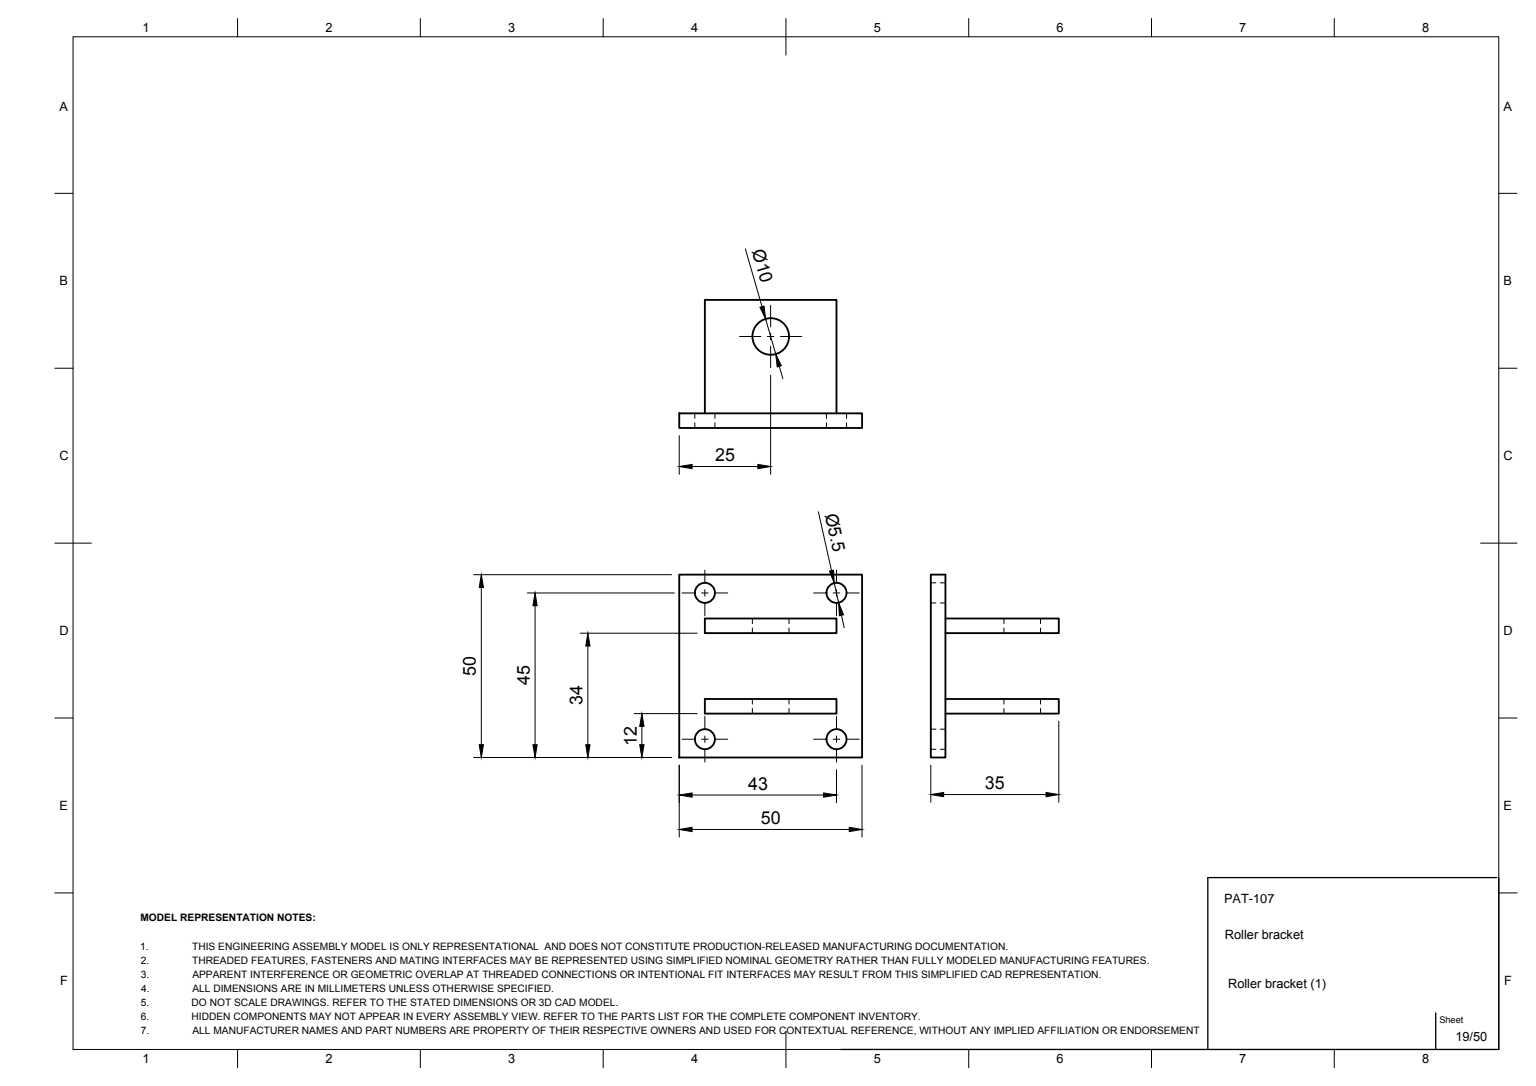
ISO-10303-21;
HEADER;
/* Generated by software containing ST-Developer
 * from STEP Tools, Inc. (www.steptools.com) 
 */

FILE_DESCRIPTION(
/* description */ ('Turntable on roller ring'),
/* implementation_level */ '2;1');

FILE_NAME(
/* name */ 'Roller bracket (1).step',
/* time_stamp */ '2026-10-28T03:23:59-07:00',
/* author */ (''),
/* organization */ (''),
/* preprocessor_version */ 'ST-DEVELOPER v20.2',
/* originating_system */ 'Autodesk Translation Framework v15.17.0.0',
/* authorisation */ '');

FILE_SCHEMA (('AUTOMOTIVE_DESIGN { 1 0 10303 214 3 1 1 }'));
ENDSEC;

DATA;
#10=MECHANICAL_DESIGN_GEOMETRIC_PRESENTATION_REPRESENTATION('',(#647),#16281);
#528=SHAPE_REPRESENTATION_RELATIONSHIP('SRR','None',#16546,#583);
#583=ADVANCED_BREP_SHAPE_REPRESENTATION('',(#717),#16240);
#647=STYLED_ITEM('',(#16911),#717);
#717=MANIFOLD_SOLID_BREP('Body1',#8390);
#889=FACE_BOUND('',#2148,.T.);
#890=FACE_BOUND('',#2150,.T.);
#891=FACE_BOUND('',#2155,.T.);
#892=FACE_BOUND('',#2157,.T.);
#893=FACE_BOUND('',#2163,.T.);
#894=FACE_BOUND('',#2164,.T.);
#895=FACE_BOUND('',#2165,.T.);
#896=FACE_BOUND('',#2166,.T.);
#897=FACE_BOUND('',#2167,.T.);
#898=FACE_BOUND('',#2168,.T.);
#899=FACE_BOUND('',#2170,.T.);
#900=FACE_BOUND('',#2171,.T.);
#901=FACE_BOUND('',#2172,.T.);
#902=FACE_BOUND('',#2173,.T.);
#1109=PLANE('',#9629);
#1110=PLANE('',#9630);
#1111=PLANE('',#9631);
#1112=PLANE('',#9632);
#1113=PLANE('',#9633);
#1114=PLANE('',#9634);
#1115=PLANE('',#9635);
#1116=PLANE('',#9636);
#1117=PLANE('',#9637);
#1118=PLANE('',#9638);
#1119=PLANE('',#9639);
#1120=PLANE('',#9640);
#1121=PLANE('',#9641);
#1122=PLANE('',#9642);
#1123=PLANE('',#9643);
#1124=PLANE('',#9644);
#1501=FACE_OUTER_BOUND('',#2138,.T.);
#1502=FACE_OUTER_BOUND('',#2139,.T.);
#1503=FACE_OUTER_BOUND('',#2140,.T.);
#1504=FACE_OUTER_BOUND('',#2141,.T.);
#1505=FACE_OUTER_BOUND('',#2142,.T.);
#1506=FACE_OUTER_BOUND('',#2143,.T.);
#1507=FACE_OUTER_BOUND('',#2144,.T.);
#1508=FACE_OUTER_BOUND('',#2145,.T.);
#1509=FACE_OUTER_BOUND('',#2146,.T.);
#1510=FACE_OUTER_BOUND('',#2147,.T.);
#1511=FACE_OUTER_BOUND('',#2149,.T.);
#1512=FACE_OUTER_BOUND('',#2151,.T.);
#1513=FACE_OUTER_BOUND('',#2152,.T.);
#1514=FACE_OUTER_BOUND('',#2153,.T.);
#1515=FACE_OUTER_BOUND('',#2154,.T.);
#1516=FACE_OUTER_BOUND('',#2156,.T.);
#1517=FACE_OUTER_BOUND('',#2158,.T.);
#1518=FACE_OUTER_BOUND('',#2159,.T.);
#1519=FACE_OUTER_BOUND('',#2160,.T.);
#1520=FACE_OUTER_BOUND('',#2161,.T.);
#1521=FACE_OUTER_BOUND('',#2162,.T.);
#1522=FACE_OUTER_BOUND('',#2169,.T.);
#2138=EDGE_LOOP('',(#6707,#6708,#6709,#6710));
#2139=EDGE_LOOP('',(#6711,#6712,#6713,#6714));
#2140=EDGE_LOOP('',(#6715,#6716,#6717,#6718));
#2141=EDGE_LOOP('',(#6719,#6720,#6721,#6722));
#2142=EDGE_LOOP('',(#6723,#6724,#6725,#6726));
#2143=EDGE_LOOP('',(#6727,#6728,#6729,#6730));
#2144=EDGE_LOOP('',(#6731,#6732,#6733,#6734));
#2145=EDGE_LOOP('',(#6735,#6736,#6737,#6738));
#2146=EDGE_LOOP('',(#6739,#6740,#6741,#6742));
#2147=EDGE_LOOP('',(#6743,#6744,#6745,#6746));
#2148=EDGE_LOOP('',(#6747));
#2149=EDGE_LOOP('',(#6748,#6749,#6750,#6751));
#2150=EDGE_LOOP('',(#6752));
#2151=EDGE_LOOP('',(#6753,#6754,#6755,#6756));
#2152=EDGE_LOOP('',(#6757,#6758,#6759,#6760));
#2153=EDGE_LOOP('',(#6761,#6762,#6763,#6764));
#2154=EDGE_LOOP('',(#6765,#6766,#6767,#6768));
#2155=EDGE_LOOP('',(#6769));
#2156=EDGE_LOOP('',(#6770,#6771,#6772,#6773));
#2157=EDGE_LOOP('',(#6774));
#2158=EDGE_LOOP('',(#6775,#6776,#6777,#6778));
#2159=EDGE_LOOP('',(#6779,#6780,#6781,#6782));
#2160=EDGE_LOOP('',(#6783,#6784,#6785,#6786));
#2161=EDGE_LOOP('',(#6787,#6788,#6789,#6790));
#2162=EDGE_LOOP('',(#6791,#6792,#6793,#6794));
#2163=EDGE_LOOP('',(#6795,#6796,#6797,#6798));
#2164=EDGE_LOOP('',(#6799,#6800,#6801,#6802));
#2165=EDGE_LOOP('',(#6803));
#2166=EDGE_LOOP('',(#6804));
#2167=EDGE_LOOP('',(#6805));
#2168=EDGE_LOOP('',(#6806));
#2169=EDGE_LOOP('',(#6807,#6808,#6809,#6810));
#2170=EDGE_LOOP('',(#6811));
#2171=EDGE_LOOP('',(#6812));
#2172=EDGE_LOOP('',(#6813));
#2173=EDGE_LOOP('',(#6814));
#2737=LINE('',#14636,#3220);
#2738=LINE('',#14642,#3221);
#2739=LINE('',#14648,#3222);
#2740=LINE('',#14654,#3223);
#2741=LINE('',#14660,#3224);
#2742=LINE('',#14666,#3225);
#2743=LINE('',#14671,#3226);
#2744=LINE('',#14673,#3227);
#2745=LINE('',#14675,#3228);
#2746=LINE('',#14676,#3229);
#2747=LINE('',#14680,#3230);
#2748=LINE('',#14682,#3231);
#2749=LINE('',#14684,#3232);
#2750=LINE('',#14685,#3233);
#2751=LINE('',#14687,#3234);
#2752=LINE('',#14688,#3235);
#2753=LINE('',#14690,#3236);
#2754=LINE('',#14692,#3237);
#2755=LINE('',#14696,#3238);
#2756=LINE('',#14698,#3239);
#2757=LINE('',#14700,#3240);
#2758=LINE('',#14701,#3241);
#2759=LINE('',#14705,#3242);
#2760=LINE('',#14707,#3243);
#2761=LINE('',#14709,#3244);
#2762=LINE('',#14710,#3245);
#2763=LINE('',#14712,#3246);
#2764=LINE('',#14713,#3247);
#2765=LINE('',#14715,#3248);
#2766=LINE('',#14717,#3249);
#2767=LINE('',#14721,#3250);
#2768=LINE('',#14723,#3251);
#2769=LINE('',#14725,#3252);
#2770=LINE('',#14726,#3253);
#2771=LINE('',#14729,#3254);
#2772=LINE('',#14731,#3255);
#2773=LINE('',#14732,#3256);
#2774=LINE('',#14735,#3257);
#2775=LINE('',#14737,#3258);
#2776=LINE('',#14738,#3259);
#2777=LINE('',#14740,#3260);
#2778=LINE('',#14741,#3261);
#3220=VECTOR('',#11590,0.275);
#3221=VECTOR('',#11597,0.275);
#3222=VECTOR('',#11604,0.275);
#3223=VECTOR('',#11611,0.275);
#3224=VECTOR('',#11618,0.5);
#3225=VECTOR('',#11625,0.5);
#3226=VECTOR('',#11630,1.);
#3227=VECTOR('',#11631,1.);
#3228=VECTOR('',#11632,1.);
#3229=VECTOR('',#11633,1.);
#3230=VECTOR('',#11636,1.);
#3231=VECTOR('',#11637,1.);
#3232=VECTOR('',#11638,1.);
#3233=VECTOR('',#11639,1.);
#3234=VECTOR('',#11642,1.);
#3235=VECTOR('',#11643,1.);
#3236=VECTOR('',#11646,1.);
#3237=VECTOR('',#11649,1.);
#3238=VECTOR('',#11652,1.);
#3239=VECTOR('',#11653,1.);
#3240=VECTOR('',#11654,1.);
#3241=VECTOR('',#11655,1.);
#3242=VECTOR('',#11658,1.);
#3243=VECTOR('',#11659,1.);
#3244=VECTOR('',#11660,1.);
#3245=VECTOR('',#11661,1.);
#3246=VECTOR('',#11664,1.);
#3247=VECTOR('',#11665,1.);
#3248=VECTOR('',#11668,1.);
#3249=VECTOR('',#11671,1.);
#3250=VECTOR('',#11674,1.);
#3251=VECTOR('',#11675,1.);
#3252=VECTOR('',#11676,1.);
#3253=VECTOR('',#11677,1.);
#3254=VECTOR('',#11680,1.);
#3255=VECTOR('',#11681,1.);
#3256=VECTOR('',#11682,1.);
#3257=VECTOR('',#11685,1.);
#3258=VECTOR('',#11686,1.);
#3259=VECTOR('',#11687,1.);
#3260=VECTOR('',#11690,1.);
#3261=VECTOR('',#11691,1.);
#3725=CIRCLE('',#9612,0.275);
#3726=CIRCLE('',#9613,0.275);
#3727=CIRCLE('',#9615,0.275);
#3728=CIRCLE('',#9616,0.275);
#3729=CIRCLE('',#9618,0.275);
#3730=CIRCLE('',#9619,0.275);
#3731=CIRCLE('',#9621,0.275);
#3732=CIRCLE('',#9622,0.275);
#3733=CIRCLE('',#9624,0.5);
#3734=CIRCLE('',#9625,0.5);
#3735=CIRCLE('',#9627,0.5);
#3736=CIRCLE('',#9628,0.5);
#4305=VERTEX_POINT('',#14633);
#4306=VERTEX_POINT('',#14635);
#4307=VERTEX_POINT('',#14639);
#4308=VERTEX_POINT('',#14641);
#4309=VERTEX_POINT('',#14645);
#4310=VERTEX_POINT('',#14647);
#4311=VERTEX_POINT('',#14651);
#4312=VERTEX_POINT('',#14653);
#4313=VERTEX_POINT('',#14657);
#4314=VERTEX_POINT('',#14659);
#4315=VERTEX_POINT('',#14663);
#4316=VERTEX_POINT('',#14665);
#4317=VERTEX_POINT('',#14669);
#4318=VERTEX_POINT('',#14670);
#4319=VERTEX_POINT('',#14672);
#4320=VERTEX_POINT('',#14674);
#4321=VERTEX_POINT('',#14678);
#4322=VERTEX_POINT('',#14679);
#4323=VERTEX_POINT('',#14681);
#4324=VERTEX_POINT('',#14683);
#4325=VERTEX_POINT('',#14694);
#4326=VERTEX_POINT('',#14695);
#4327=VERTEX_POINT('',#14697);
#4328=VERTEX_POINT('',#14699);
#4329=VERTEX_POINT('',#14703);
#4330=VERTEX_POINT('',#14704);
#4331=VERTEX_POINT('',#14706);
#4332=VERTEX_POINT('',#14708);
#4333=VERTEX_POINT('',#14719);
#4334=VERTEX_POINT('',#14720);
#4335=VERTEX_POINT('',#14722);
#4336=VERTEX_POINT('',#14724);
#4337=VERTEX_POINT('',#14728);
#4338=VERTEX_POINT('',#14730);
#4339=VERTEX_POINT('',#14734);
#4340=VERTEX_POINT('',#14736);
#5164=EDGE_CURVE('',#4305,#4305,#3725,.T.);
#5165=EDGE_CURVE('',#4305,#4306,#2737,.T.);
#5166=EDGE_CURVE('',#4306,#4306,#3726,.T.);
#5167=EDGE_CURVE('',#4307,#4307,#3727,.T.);
#5168=EDGE_CURVE('',#4307,#4308,#2738,.T.);
#5169=EDGE_CURVE('',#4308,#4308,#3728,.T.);
#5170=EDGE_CURVE('',#4309,#4309,#3729,.T.);
#5171=EDGE_CURVE('',#4309,#4310,#2739,.T.);
#5172=EDGE_CURVE('',#4310,#4310,#3730,.T.);
#5173=EDGE_CURVE('',#4311,#4311,#3731,.T.);
#5174=EDGE_CURVE('',#4311,#4312,#2740,.T.);
#5175=EDGE_CURVE('',#4312,#4312,#3732,.T.);
#5176=EDGE_CURVE('',#4313,#4313,#3733,.T.);
#5177=EDGE_CURVE('',#4313,#4314,#2741,.T.);
#5178=EDGE_CURVE('',#4314,#4314,#3734,.T.);
#5179=EDGE_CURVE('',#4315,#4315,#3735,.T.);
#5180=EDGE_CURVE('',#4315,#4316,#2742,.T.);
#5181=EDGE_CURVE('',#4316,#4316,#3736,.T.);
#5182=EDGE_CURVE('',#4317,#4318,#2743,.T.);
#5183=EDGE_CURVE('',#4317,#4319,#2744,.T.);
#5184=EDGE_CURVE('',#4320,#4319,#2745,.T.);
#5185=EDGE_CURVE('',#4318,#4320,#2746,.T.);
#5186=EDGE_CURVE('',#4321,#4322,#2747,.T.);
#5187=EDGE_CURVE('',#4323,#4321,#2748,.T.);
#5188=EDGE_CURVE('',#4324,#4323,#2749,.T.);
#5189=EDGE_CURVE('',#4322,#4324,#2750,.T.);
#5190=EDGE_CURVE('',#4322,#4317,#2751,.T.);
#5191=EDGE_CURVE('',#4319,#4324,#2752,.T.);
#5192=EDGE_CURVE('',#4320,#4323,#2753,.T.);
#5193=EDGE_CURVE('',#4321,#4318,#2754,.T.);
#5194=EDGE_CURVE('',#4325,#4326,#2755,.T.);
#5195=EDGE_CURVE('',#4325,#4327,#2756,.T.);
#5196=EDGE_CURVE('',#4328,#4327,#2757,.T.);
#5197=EDGE_CURVE('',#4326,#4328,#2758,.T.);
#5198=EDGE_CURVE('',#4329,#4330,#2759,.T.);
#5199=EDGE_CURVE('',#4331,#4329,#2760,.T.);
#5200=EDGE_CURVE('',#4332,#4331,#2761,.T.);
#5201=EDGE_CURVE('',#4330,#4332,#2762,.T.);
#5202=EDGE_CURVE('',#4330,#4325,#2763,.T.);
#5203=EDGE_CURVE('',#4327,#4332,#2764,.T.);
#5204=EDGE_CURVE('',#4328,#4331,#2765,.T.);
#5205=EDGE_CURVE('',#4329,#4326,#2766,.T.);
#5206=EDGE_CURVE('',#4333,#4334,#2767,.T.);
#5207=EDGE_CURVE('',#4334,#4335,#2768,.T.);
#5208=EDGE_CURVE('',#4336,#4335,#2769,.T.);
#5209=EDGE_CURVE('',#4333,#4336,#2770,.T.);
#5210=EDGE_CURVE('',#4337,#4333,#2771,.T.);
#5211=EDGE_CURVE('',#4338,#4336,#2772,.T.);
#5212=EDGE_CURVE('',#4337,#4338,#2773,.T.);
#5213=EDGE_CURVE('',#4339,#4337,#2774,.T.);
#5214=EDGE_CURVE('',#4340,#4338,#2775,.T.);
#5215=EDGE_CURVE('',#4339,#4340,#2776,.T.);
#5216=EDGE_CURVE('',#4334,#4339,#2777,.T.);
#5217=EDGE_CURVE('',#4335,#4340,#2778,.T.);
#6707=ORIENTED_EDGE('',*,*,#5164,.F.);
#6708=ORIENTED_EDGE('',*,*,#5165,.T.);
#6709=ORIENTED_EDGE('',*,*,#5166,.F.);
#6710=ORIENTED_EDGE('',*,*,#5165,.F.);
#6711=ORIENTED_EDGE('',*,*,#5167,.F.);
#6712=ORIENTED_EDGE('',*,*,#5168,.T.);
#6713=ORIENTED_EDGE('',*,*,#5169,.F.);
#6714=ORIENTED_EDGE('',*,*,#5168,.F.);
#6715=ORIENTED_EDGE('',*,*,#5170,.F.);
#6716=ORIENTED_EDGE('',*,*,#5171,.T.);
#6717=ORIENTED_EDGE('',*,*,#5172,.F.);
#6718=ORIENTED_EDGE('',*,*,#5171,.F.);
#6719=ORIENTED_EDGE('',*,*,#5173,.F.);
#6720=ORIENTED_EDGE('',*,*,#5174,.T.);
#6721=ORIENTED_EDGE('',*,*,#5175,.F.);
#6722=ORIENTED_EDGE('',*,*,#5174,.F.);
#6723=ORIENTED_EDGE('',*,*,#5176,.F.);
#6724=ORIENTED_EDGE('',*,*,#5177,.T.);
#6725=ORIENTED_EDGE('',*,*,#5178,.F.);
#6726=ORIENTED_EDGE('',*,*,#5177,.F.);
#6727=ORIENTED_EDGE('',*,*,#5179,.F.);
#6728=ORIENTED_EDGE('',*,*,#5180,.T.);
#6729=ORIENTED_EDGE('',*,*,#5181,.F.);
#6730=ORIENTED_EDGE('',*,*,#5180,.F.);
#6731=ORIENTED_EDGE('',*,*,#5182,.F.);
#6732=ORIENTED_EDGE('',*,*,#5183,.T.);
#6733=ORIENTED_EDGE('',*,*,#5184,.F.);
#6734=ORIENTED_EDGE('',*,*,#5185,.F.);
#6735=ORIENTED_EDGE('',*,*,#5186,.F.);
#6736=ORIENTED_EDGE('',*,*,#5187,.F.);
#6737=ORIENTED_EDGE('',*,*,#5188,.F.);
#6738=ORIENTED_EDGE('',*,*,#5189,.F.);
#6739=ORIENTED_EDGE('',*,*,#5190,.F.);
#6740=ORIENTED_EDGE('',*,*,#5189,.T.);
#6741=ORIENTED_EDGE('',*,*,#5191,.F.);
#6742=ORIENTED_EDGE('',*,*,#5183,.F.);
#6743=ORIENTED_EDGE('',*,*,#5191,.T.);
#6744=ORIENTED_EDGE('',*,*,#5188,.T.);
#6745=ORIENTED_EDGE('',*,*,#5192,.F.);
#6746=ORIENTED_EDGE('',*,*,#5184,.T.);
#6747=ORIENTED_EDGE('',*,*,#5181,.T.);
#6748=ORIENTED_EDGE('',*,*,#5190,.T.);
#6749=ORIENTED_EDGE('',*,*,#5182,.T.);
#6750=ORIENTED_EDGE('',*,*,#5193,.F.);
#6751=ORIENTED_EDGE('',*,*,#5186,.T.);
#6752=ORIENTED_EDGE('',*,*,#5179,.T.);
#6753=ORIENTED_EDGE('',*,*,#5194,.F.);
#6754=ORIENTED_EDGE('',*,*,#5195,.T.);
#6755=ORIENTED_EDGE('',*,*,#5196,.F.);
#6756=ORIENTED_EDGE('',*,*,#5197,.F.);
#6757=ORIENTED_EDGE('',*,*,#5198,.F.);
#6758=ORIENTED_EDGE('',*,*,#5199,.F.);
#6759=ORIENTED_EDGE('',*,*,#5200,.F.);
#6760=ORIENTED_EDGE('',*,*,#5201,.F.);
#6761=ORIENTED_EDGE('',*,*,#5202,.F.);
#6762=ORIENTED_EDGE('',*,*,#5201,.T.);
#6763=ORIENTED_EDGE('',*,*,#5203,.F.);
#6764=ORIENTED_EDGE('',*,*,#5195,.F.);
#6765=ORIENTED_EDGE('',*,*,#5203,.T.);
#6766=ORIENTED_EDGE('',*,*,#5200,.T.);
#6767=ORIENTED_EDGE('',*,*,#5204,.F.);
#6768=ORIENTED_EDGE('',*,*,#5196,.T.);
#6769=ORIENTED_EDGE('',*,*,#5178,.T.);
#6770=ORIENTED_EDGE('',*,*,#5202,.T.);
#6771=ORIENTED_EDGE('',*,*,#5194,.T.);
#6772=ORIENTED_EDGE('',*,*,#5205,.F.);
#6773=ORIENTED_EDGE('',*,*,#5198,.T.);
#6774=ORIENTED_EDGE('',*,*,#5176,.T.);
#6775=ORIENTED_EDGE('',*,*,#5206,.T.);
#6776=ORIENTED_EDGE('',*,*,#5207,.T.);
#6777=ORIENTED_EDGE('',*,*,#5208,.F.);
#6778=ORIENTED_EDGE('',*,*,#5209,.F.);
#6779=ORIENTED_EDGE('',*,*,#5210,.T.);
#6780=ORIENTED_EDGE('',*,*,#5209,.T.);
#6781=ORIENTED_EDGE('',*,*,#5211,.F.);
#6782=ORIENTED_EDGE('',*,*,#5212,.F.);
#6783=ORIENTED_EDGE('',*,*,#5213,.T.);
#6784=ORIENTED_EDGE('',*,*,#5212,.T.);
#6785=ORIENTED_EDGE('',*,*,#5214,.F.);
#6786=ORIENTED_EDGE('',*,*,#5215,.F.);
#6787=ORIENTED_EDGE('',*,*,#5216,.T.);
#6788=ORIENTED_EDGE('',*,*,#5215,.T.);
#6789=ORIENTED_EDGE('',*,*,#5217,.F.);
#6790=ORIENTED_EDGE('',*,*,#5207,.F.);
#6791=ORIENTED_EDGE('',*,*,#5217,.T.);
#6792=ORIENTED_EDGE('',*,*,#5214,.T.);
#6793=ORIENTED_EDGE('',*,*,#5211,.T.);
#6794=ORIENTED_EDGE('',*,*,#5208,.T.);
#6795=ORIENTED_EDGE('',*,*,#5199,.T.);
#6796=ORIENTED_EDGE('',*,*,#5205,.T.);
#6797=ORIENTED_EDGE('',*,*,#5197,.T.);
#6798=ORIENTED_EDGE('',*,*,#5204,.T.);
#6799=ORIENTED_EDGE('',*,*,#5187,.T.);
#6800=ORIENTED_EDGE('',*,*,#5193,.T.);
#6801=ORIENTED_EDGE('',*,*,#5185,.T.);
#6802=ORIENTED_EDGE('',*,*,#5192,.T.);
#6803=ORIENTED_EDGE('',*,*,#5175,.T.);
#6804=ORIENTED_EDGE('',*,*,#5172,.T.);
#6805=ORIENTED_EDGE('',*,*,#5169,.T.);
#6806=ORIENTED_EDGE('',*,*,#5166,.T.);
#6807=ORIENTED_EDGE('',*,*,#5216,.F.);
#6808=ORIENTED_EDGE('',*,*,#5206,.F.);
#6809=ORIENTED_EDGE('',*,*,#5210,.F.);
#6810=ORIENTED_EDGE('',*,*,#5213,.F.);
#6811=ORIENTED_EDGE('',*,*,#5164,.T.);
#6812=ORIENTED_EDGE('',*,*,#5167,.T.);
#6813=ORIENTED_EDGE('',*,*,#5170,.T.);
#6814=ORIENTED_EDGE('',*,*,#5173,.T.);
#7768=CYLINDRICAL_SURFACE('',#9611,0.275);
#7769=CYLINDRICAL_SURFACE('',#9614,0.275);
#7770=CYLINDRICAL_SURFACE('',#9617,0.275);
#7771=CYLINDRICAL_SURFACE('',#9620,0.275);
#7772=CYLINDRICAL_SURFACE('',#9623,0.5);
#7773=CYLINDRICAL_SURFACE('',#9626,0.5);
#8104=ADVANCED_FACE('',(#1501),#7768,.F.);
#8105=ADVANCED_FACE('',(#1502),#7769,.F.);
#8106=ADVANCED_FACE('',(#1503),#7770,.F.);
#8107=ADVANCED_FACE('',(#1504),#7771,.F.);
#8108=ADVANCED_FACE('',(#1505),#7772,.F.);
#8109=ADVANCED_FACE('',(#1506),#7773,.F.);
#8110=ADVANCED_FACE('',(#1507),#1109,.T.);
#8111=ADVANCED_FACE('',(#1508),#1110,.T.);
#8112=ADVANCED_FACE('',(#1509),#1111,.T.);
#8113=ADVANCED_FACE('',(#1510,#889),#1112,.T.);
#8114=ADVANCED_FACE('',(#1511,#890),#1113,.F.);
#8115=ADVANCED_FACE('',(#1512),#1114,.T.);
#8116=ADVANCED_FACE('',(#1513),#1115,.T.);
#8117=ADVANCED_FACE('',(#1514),#1116,.T.);
#8118=ADVANCED_FACE('',(#1515,#891),#1117,.T.);
#8119=ADVANCED_FACE('',(#1516,#892),#1118,.F.);
#8120=ADVANCED_FACE('',(#1517),#1119,.T.);
#8121=ADVANCED_FACE('',(#1518),#1120,.T.);
#8122=ADVANCED_FACE('',(#1519),#1121,.T.);
#8123=ADVANCED_FACE('',(#1520),#1122,.T.);
#8124=ADVANCED_FACE('',(#1521,#893,#894,#895,#896,#897,#898),#1123,.T.);
#8125=ADVANCED_FACE('',(#1522,#899,#900,#901,#902),#1124,.F.);
#8390=CLOSED_SHELL('',(#8104,#8105,#8106,#8107,#8108,#8109,#8110,#8111,
#8112,#8113,#8114,#8115,#8116,#8117,#8118,#8119,#8120,#8121,#8122,#8123,
#8124,#8125));
#9610=AXIS2_PLACEMENT_3D('',#14631,#11584,#11585);
#9611=AXIS2_PLACEMENT_3D('',#14632,#11586,#11587);
#9612=AXIS2_PLACEMENT_3D('',#14634,#11588,#11589);
#9613=AXIS2_PLACEMENT_3D('',#14637,#11591,#11592);
#9614=AXIS2_PLACEMENT_3D('',#14638,#11593,#11594);
#9615=AXIS2_PLACEMENT_3D('',#14640,#11595,#11596);
#9616=AXIS2_PLACEMENT_3D('',#14643,#11598,#11599);
#9617=AXIS2_PLACEMENT_3D('',#14644,#11600,#11601);
#9618=AXIS2_PLACEMENT_3D('',#14646,#11602,#11603);
#9619=AXIS2_PLACEMENT_3D('',#14649,#11605,#11606);
#9620=AXIS2_PLACEMENT_3D('',#14650,#11607,#11608);
#9621=AXIS2_PLACEMENT_3D('',#14652,#11609,#11610);
#9622=AXIS2_PLACEMENT_3D('',#14655,#11612,#11613);
#9623=AXIS2_PLACEMENT_3D('',#14656,#11614,#11615);
#9624=AXIS2_PLACEMENT_3D('',#14658,#11616,#11617);
#9625=AXIS2_PLACEMENT_3D('',#14661,#11619,#11620);
#9626=AXIS2_PLACEMENT_3D('',#14662,#11621,#11622);
#9627=AXIS2_PLACEMENT_3D('',#14664,#11623,#11624);
#9628=AXIS2_PLACEMENT_3D('',#14667,#11626,#11627);
#9629=AXIS2_PLACEMENT_3D('',#14668,#11628,#11629);
#9630=AXIS2_PLACEMENT_3D('',#14677,#11634,#11635);
#9631=AXIS2_PLACEMENT_3D('',#14686,#11640,#11641);
#9632=AXIS2_PLACEMENT_3D('',#14689,#11644,#11645);
#9633=AXIS2_PLACEMENT_3D('',#14691,#11647,#11648);
#9634=AXIS2_PLACEMENT_3D('',#14693,#11650,#11651);
#9635=AXIS2_PLACEMENT_3D('',#14702,#11656,#11657);
#9636=AXIS2_PLACEMENT_3D('',#14711,#11662,#11663);
#9637=AXIS2_PLACEMENT_3D('',#14714,#11666,#11667);
#9638=AXIS2_PLACEMENT_3D('',#14716,#11669,#11670);
#9639=AXIS2_PLACEMENT_3D('',#14718,#11672,#11673);
#9640=AXIS2_PLACEMENT_3D('',#14727,#11678,#11679);
#9641=AXIS2_PLACEMENT_3D('',#14733,#11683,#11684);
#9642=AXIS2_PLACEMENT_3D('',#14739,#11688,#11689);
#9643=AXIS2_PLACEMENT_3D('',#14742,#11692,#11693);
#9644=AXIS2_PLACEMENT_3D('',#14743,#11694,#11695);
#11584=DIRECTION('axis',(0.,0.,1.));
#11585=DIRECTION('refdir',(1.,0.,0.));
#11586=DIRECTION('center_axis',(0.,0.,1.));
#11587=DIRECTION('ref_axis',(1.,0.,0.));
#11588=DIRECTION('center_axis',(0.,0.,1.));
#11589=DIRECTION('ref_axis',(1.,0.,0.));
#11590=DIRECTION('',(0.,0.,1.));
#11591=DIRECTION('center_axis',(0.,0.,-1.));
#11592=DIRECTION('ref_axis',(1.,0.,0.));
#11593=DIRECTION('center_axis',(0.,0.,1.));
#11594=DIRECTION('ref_axis',(1.,0.,0.));
#11595=DIRECTION('center_axis',(0.,0.,1.));
#11596=DIRECTION('ref_axis',(1.,0.,0.));
#11597=DIRECTION('',(0.,0.,1.));
#11598=DIRECTION('center_axis',(0.,0.,-1.));
#11599=DIRECTION('ref_axis',(1.,0.,0.));
#11600=DIRECTION('center_axis',(0.,0.,1.));
#11601=DIRECTION('ref_axis',(1.,0.,0.));
#11602=DIRECTION('center_axis',(0.,0.,1.));
#11603=DIRECTION('ref_axis',(1.,0.,0.));
#11604=DIRECTION('',(0.,0.,1.));
#11605=DIRECTION('center_axis',(0.,0.,-1.));
#11606=DIRECTION('ref_axis',(1.,0.,0.));
#11607=DIRECTION('center_axis',(0.,0.,1.));
#11608=DIRECTION('ref_axis',(1.,0.,0.));
#11609=DIRECTION('center_axis',(0.,0.,1.));
#11610=DIRECTION('ref_axis',(1.,0.,0.));
#11611=DIRECTION('',(0.,0.,1.));
#11612=DIRECTION('center_axis',(0.,0.,-1.));
#11613=DIRECTION('ref_axis',(1.,0.,0.));
#11614=DIRECTION('center_axis',(0.,1.,0.));
#11615=DIRECTION('ref_axis',(1.,0.,0.));
#11616=DIRECTION('center_axis',(0.,1.,0.));
#11617=DIRECTION('ref_axis',(1.,0.,0.));
#11618=DIRECTION('',(0.,1.,0.));
#11619=DIRECTION('center_axis',(0.,-1.,0.));
#11620=DIRECTION('ref_axis',(1.,0.,0.));
#11621=DIRECTION('center_axis',(0.,1.,0.));
#11622=DIRECTION('ref_axis',(1.,0.,0.));
#11623=DIRECTION('center_axis',(0.,1.,0.));
#11624=DIRECTION('ref_axis',(1.,0.,0.));
#11625=DIRECTION('',(0.,1.,0.));
#11626=DIRECTION('center_axis',(0.,-1.,0.));
#11627=DIRECTION('ref_axis',(1.,0.,0.));
#11628=DIRECTION('center_axis',(-1.,0.,0.));
#11629=DIRECTION('ref_axis',(0.,0.,1.));
#11630=DIRECTION('',(0.,0.,-1.));
#11631=DIRECTION('',(0.,1.,0.));
#11632=DIRECTION('',(0.,0.,1.));
#11633=DIRECTION('',(0.,1.,0.));
#11634=DIRECTION('center_axis',(1.,0.,0.));
#11635=DIRECTION('ref_axis',(0.,0.,-1.));
#11636=DIRECTION('',(0.,0.,1.));
#11637=DIRECTION('',(0.,-1.,0.));
#11638=DIRECTION('',(0.,0.,-1.));
#11639=DIRECTION('',(0.,1.,0.));
#11640=DIRECTION('center_axis',(0.,0.,1.));
#11641=DIRECTION('ref_axis',(1.,0.,0.));
#11642=DIRECTION('',(-1.,0.,0.));
#11643=DIRECTION('',(1.,0.,0.));
#11644=DIRECTION('center_axis',(0.,1.,0.));
#11645=DIRECTION('ref_axis',(0.,0.,1.));
#11646=DIRECTION('',(1.,0.,0.));
#11647=DIRECTION('center_axis',(0.,1.,0.));
#11648=DIRECTION('ref_axis',(1.,0.,0.));
#11649=DIRECTION('',(-1.,0.,0.));
#11650=DIRECTION('center_axis',(-1.,0.,0.));
#11651=DIRECTION('ref_axis',(0.,0.,1.));
#11652=DIRECTION('',(0.,0.,-1.));
#11653=DIRECTION('',(0.,1.,0.));
#11654=DIRECTION('',(0.,0.,1.));
#11655=DIRECTION('',(0.,1.,0.));
#11656=DIRECTION('center_axis',(1.,0.,0.));
#11657=DIRECTION('ref_axis',(0.,0.,-1.));
#11658=DIRECTION('',(0.,0.,1.));
#11659=DIRECTION('',(0.,-1.,0.));
#11660=DIRECTION('',(0.,0.,-1.));
#11661=DIRECTION('',(0.,1.,0.));
#11662=DIRECTION('center_axis',(0.,0.,1.));
#11663=DIRECTION('ref_axis',(1.,0.,0.));
#11664=DIRECTION('',(-1.,0.,0.));
#11665=DIRECTION('',(1.,0.,0.));
#11666=DIRECTION('center_axis',(0.,1.,0.));
#11667=DIRECTION('ref_axis',(0.,0.,1.));
#11668=DIRECTION('',(1.,0.,0.));
#11669=DIRECTION('center_axis',(0.,1.,0.));
#11670=DIRECTION('ref_axis',(1.,0.,0.));
#11671=DIRECTION('',(-1.,0.,0.));
#11672=DIRECTION('center_axis',(0.,1.,0.));
#11673=DIRECTION('ref_axis',(-1.,0.,0.));
#11674=DIRECTION('',(-1.,0.,0.));
#11675=DIRECTION('',(0.,0.,1.));
#11676=DIRECTION('',(-1.,0.,0.));
#11677=DIRECTION('',(0.,0.,1.));
#11678=DIRECTION('center_axis',(1.,0.,0.));
#11679=DIRECTION('ref_axis',(0.,1.,0.));
#11680=DIRECTION('',(0.,1.,0.));
#11681=DIRECTION('',(0.,1.,0.));
#11682=DIRECTION('',(0.,0.,1.));
#11683=DIRECTION('center_axis',(0.,-1.,0.));
#11684=DIRECTION('ref_axis',(1.,0.,0.));
#11685=DIRECTION('',(1.,0.,0.));
#11686=DIRECTION('',(1.,0.,0.));
#11687=DIRECTION('',(0.,0.,1.));
#11688=DIRECTION('center_axis',(-1.,0.,0.));
#11689=DIRECTION('ref_axis',(0.,-1.,0.));
#11690=DIRECTION('',(0.,-1.,0.));
#11691=DIRECTION('',(0.,-1.,0.));
#11692=DIRECTION('center_axis',(0.,0.,1.));
#11693=DIRECTION('ref_axis',(1.,0.,0.));
#11694=DIRECTION('center_axis',(0.,0.,1.));
#11695=DIRECTION('ref_axis',(1.,0.,0.));
#14631=CARTESIAN_POINT('',(0.,0.,0.));
#14632=CARTESIAN_POINT('Origin',(1.8,13.,0.9));
#14633=CARTESIAN_POINT('',(1.525,13.,1.));
#14634=CARTESIAN_POINT('Origin',(1.8,13.,1.));
#14635=CARTESIAN_POINT('',(1.525,13.,1.4));
#14636=CARTESIAN_POINT('',(1.525,13.,0.9));
#14637=CARTESIAN_POINT('Origin',(1.8,13.,1.4));
#14638=CARTESIAN_POINT('Origin',(-1.8,17.,0.9));
#14639=CARTESIAN_POINT('',(-2.075,17.,1.));
#14640=CARTESIAN_POINT('Origin',(-1.8,17.,1.));
#14641=CARTESIAN_POINT('',(-2.075,17.,1.4));
#14642=CARTESIAN_POINT('',(-2.075,17.,0.9));
#14643=CARTESIAN_POINT('Origin',(-1.8,17.,1.4));
#14644=CARTESIAN_POINT('Origin',(-1.8,13.,0.9));
#14645=CARTESIAN_POINT('',(-2.075,13.,1.));
#14646=CARTESIAN_POINT('Origin',(-1.8,13.,1.));
#14647=CARTESIAN_POINT('',(-2.075,13.,1.4));
#14648=CARTESIAN_POINT('',(-2.075,13.,0.9));
#14649=CARTESIAN_POINT('Origin',(-1.8,13.,1.4));
#14650=CARTESIAN_POINT('Origin',(1.8,17.,0.9));
#14651=CARTESIAN_POINT('',(1.525,17.,1.));
#14652=CARTESIAN_POINT('Origin',(1.8,17.,1.));
#14653=CARTESIAN_POINT('',(1.525,17.,1.4));
#14654=CARTESIAN_POINT('',(1.525,17.,0.9));
#14655=CARTESIAN_POINT('Origin',(1.8,17.,1.4));
#14656=CARTESIAN_POINT('Origin',(0.,13.6,3.5));
#14657=CARTESIAN_POINT('',(-0.5,13.7,3.5));
#14658=CARTESIAN_POINT('Origin',(0.,13.7,3.5));
#14659=CARTESIAN_POINT('',(-0.5,14.1,3.5));
#14660=CARTESIAN_POINT('',(-0.5,13.6,3.5));
#14661=CARTESIAN_POINT('Origin',(0.,14.1,3.5));
#14662=CARTESIAN_POINT('Origin',(0.,13.6,3.5));
#14663=CARTESIAN_POINT('',(-0.5,15.9,3.5));
#14664=CARTESIAN_POINT('Origin',(0.,15.9,3.5));
#14665=CARTESIAN_POINT('',(-0.5,16.3,3.5));
#14666=CARTESIAN_POINT('',(-0.5,13.6,3.5));
#14667=CARTESIAN_POINT('Origin',(0.,16.3,3.5));
#14668=CARTESIAN_POINT('Origin',(-1.8,15.9,1.4));
#14669=CARTESIAN_POINT('',(-1.8,15.9,4.5));
#14670=CARTESIAN_POINT('',(-1.8,15.9,1.4));
#14671=CARTESIAN_POINT('',(-1.8,15.9,4.5));
#14672=CARTESIAN_POINT('',(-1.8,16.3,4.5));
#14673=CARTESIAN_POINT('',(-1.8,15.9,4.5));
#14674=CARTESIAN_POINT('',(-1.8,16.3,1.4));
#14675=CARTESIAN_POINT('',(-1.8,16.3,4.5));
#14676=CARTESIAN_POINT('',(-1.8,15.45,1.4));
#14677=CARTESIAN_POINT('Origin',(1.8,15.9,4.5));
#14678=CARTESIAN_POINT('',(1.8,15.9,1.4));
#14679=CARTESIAN_POINT('',(1.8,15.9,4.5));
#14680=CARTESIAN_POINT('',(1.8,15.9,1.4));
#14681=CARTESIAN_POINT('',(1.8,16.3,1.4));
#14682=CARTESIAN_POINT('',(1.8,15.45,1.4));
#14683=CARTESIAN_POINT('',(1.8,16.3,4.5));
#14684=CARTESIAN_POINT('',(1.8,16.3,1.4));
#14685=CARTESIAN_POINT('',(1.8,15.9,4.5));
#14686=CARTESIAN_POINT('Origin',(-1.8,15.9,4.5));
#14687=CARTESIAN_POINT('',(1.8,15.9,4.5));
#14688=CARTESIAN_POINT('',(1.8,16.3,4.5));
#14689=CARTESIAN_POINT('Origin',(0.,16.3,2.95));
#14690=CARTESIAN_POINT('',(0.,16.3,1.4));
#14691=CARTESIAN_POINT('Origin',(0.,15.9,2.95));
#14692=CARTESIAN_POINT('',(0.,15.9,1.4));
#14693=CARTESIAN_POINT('Origin',(-1.8,13.7,1.4));
#14694=CARTESIAN_POINT('',(-1.8,13.7,4.5));
#14695=CARTESIAN_POINT('',(-1.8,13.7,1.4));
#14696=CARTESIAN_POINT('',(-1.8,13.7,4.5));
#14697=CARTESIAN_POINT('',(-1.8,14.1,4.5));
#14698=CARTESIAN_POINT('',(-1.8,13.7,4.5));
#14699=CARTESIAN_POINT('',(-1.8,14.1,1.4));
#14700=CARTESIAN_POINT('',(-1.8,14.1,4.5));
#14701=CARTESIAN_POINT('',(-1.8,14.35,1.4));
#14702=CARTESIAN_POINT('Origin',(1.8,13.7,4.5));
#14703=CARTESIAN_POINT('',(1.8,13.7,1.4));
#14704=CARTESIAN_POINT('',(1.8,13.7,4.5));
#14705=CARTESIAN_POINT('',(1.8,13.7,1.4));
#14706=CARTESIAN_POINT('',(1.8,14.1,1.4));
#14707=CARTESIAN_POINT('',(1.8,14.35,1.4));
#14708=CARTESIAN_POINT('',(1.8,14.1,4.5));
#14709=CARTESIAN_POINT('',(1.8,14.1,1.4));
#14710=CARTESIAN_POINT('',(1.8,13.7,4.5));
#14711=CARTESIAN_POINT('Origin',(-1.8,13.7,4.5));
#14712=CARTESIAN_POINT('',(1.8,13.7,4.5));
#14713=CARTESIAN_POINT('',(1.8,14.1,4.5));
#14714=CARTESIAN_POINT('Origin',(0.,14.1,2.95));
#14715=CARTESIAN_POINT('',(0.,14.1,1.4));
#14716=CARTESIAN_POINT('Origin',(0.,13.7,2.95));
#14717=CARTESIAN_POINT('',(0.,13.7,1.4));
#14718=CARTESIAN_POINT('Origin',(2.5,17.5,1.));
#14719=CARTESIAN_POINT('',(2.5,17.5,1.));
#14720=CARTESIAN_POINT('',(-2.5,17.5,1.));
#14721=CARTESIAN_POINT('',(2.5,17.5,1.));
#14722=CARTESIAN_POINT('',(-2.5,17.5,1.4));
#14723=CARTESIAN_POINT('',(-2.5,17.5,1.));
#14724=CARTESIAN_POINT('',(2.5,17.5,1.4));
#14725=CARTESIAN_POINT('',(2.5,17.5,1.4));
#14726=CARTESIAN_POINT('',(2.5,17.5,1.));
#14727=CARTESIAN_POINT('Origin',(2.5,12.5,1.));
#14728=CARTESIAN_POINT('',(2.5,12.5,1.));
#14729=CARTESIAN_POINT('',(2.5,12.5,1.));
#14730=CARTESIAN_POINT('',(2.5,12.5,1.4));
#14731=CARTESIAN_POINT('',(2.5,12.5,1.4));
#14732=CARTESIAN_POINT('',(2.5,12.5,1.));
#14733=CARTESIAN_POINT('Origin',(-2.5,12.5,1.));
#14734=CARTESIAN_POINT('',(-2.5,12.5,1.));
#14735=CARTESIAN_POINT('',(-2.5,12.5,1.));
#14736=CARTESIAN_POINT('',(-2.5,12.5,1.4));
#14737=CARTESIAN_POINT('',(-2.5,12.5,1.4));
#14738=CARTESIAN_POINT('',(-2.5,12.5,1.));
#14739=CARTESIAN_POINT('Origin',(-2.5,17.5,1.));
#14740=CARTESIAN_POINT('',(-2.5,17.5,1.));
#14741=CARTESIAN_POINT('',(-2.5,17.5,1.4));
#14742=CARTESIAN_POINT('Origin',(0.,15.,1.4));
#14743=CARTESIAN_POINT('Origin',(0.,15.,1.));
#16171=UNCERTAINTY_MEASURE_WITH_UNIT(LENGTH_MEASURE(0.001),#16282,
'DISTANCE_ACCURACY_VALUE',
'Maximum model space distance between geometric entities at asserted c
onnectivities');
#16212=UNCERTAINTY_MEASURE_WITH_UNIT(LENGTH_MEASURE(0.001),#16282,
'DISTANCE_ACCURACY_VALUE',
'Maximum model space distance between geometric entities at asserted c
onnectivities');
#16240=(
GEOMETRIC_REPRESENTATION_CONTEXT(3)
GLOBAL_UNCERTAINTY_ASSIGNED_CONTEXT((#16171))
GLOBAL_UNIT_ASSIGNED_CONTEXT((#16282,#16284,#16285))
REPRESENTATION_CONTEXT('','3D')
);
#16281=(
GEOMETRIC_REPRESENTATION_CONTEXT(3)
GLOBAL_UNCERTAINTY_ASSIGNED_CONTEXT((#16212))
GLOBAL_UNIT_ASSIGNED_CONTEXT((#16282,#16284,#16285))
REPRESENTATION_CONTEXT('','3D')
);
#16282=(
LENGTH_UNIT()
NAMED_UNIT(*)
SI_UNIT(.CENTI.,.METRE.)
);
#16284=(
NAMED_UNIT(*)
PLANE_ANGLE_UNIT()
SI_UNIT($,.RADIAN.)
);
#16285=(
NAMED_UNIT(*)
SI_UNIT($,.STERADIAN.)
SOLID_ANGLE_UNIT()
);
#16313=SHAPE_DEFINITION_REPRESENTATION(#16407,#16546);
#16407=PRODUCT_DEFINITION_SHAPE('',$,#16615);
#16546=SHAPE_REPRESENTATION('',(#9610),#16240);
#16587=PRODUCT_DEFINITION_CONTEXT('part definition',#16793,'design');
#16615=PRODUCT_DEFINITION('Roller bracket (1)','Roller bracket (1)',#16683,
#16587);
#16683=PRODUCT_DEFINITION_FORMATION('',$,#16822);
#16793=APPLICATION_CONTEXT(
'Core Data for Automotive Mechanical Design Process');
#16794=PRODUCT_CONTEXT('part definition',#16793,'mechanical');
#16822=PRODUCT('Roller bracket (1)','Roller bracket (1)','Roller bracket (1)',
(#16794));
#16905=COLOUR_RGB('Dark Blue',0.08,0.2,0.34);
#16906=FILL_AREA_STYLE_COLOUR('',#16905);
#16907=FILL_AREA_STYLE('',(#16906));
#16908=SURFACE_STYLE_FILL_AREA(#16907);
#16909=SURFACE_SIDE_STYLE('',(#16908));
#16910=SURFACE_STYLE_USAGE(.BOTH.,#16909);
#16911=PRESENTATION_STYLE_ASSIGNMENT((#16910));
ENDSEC;
END-ISO-10303-21;
